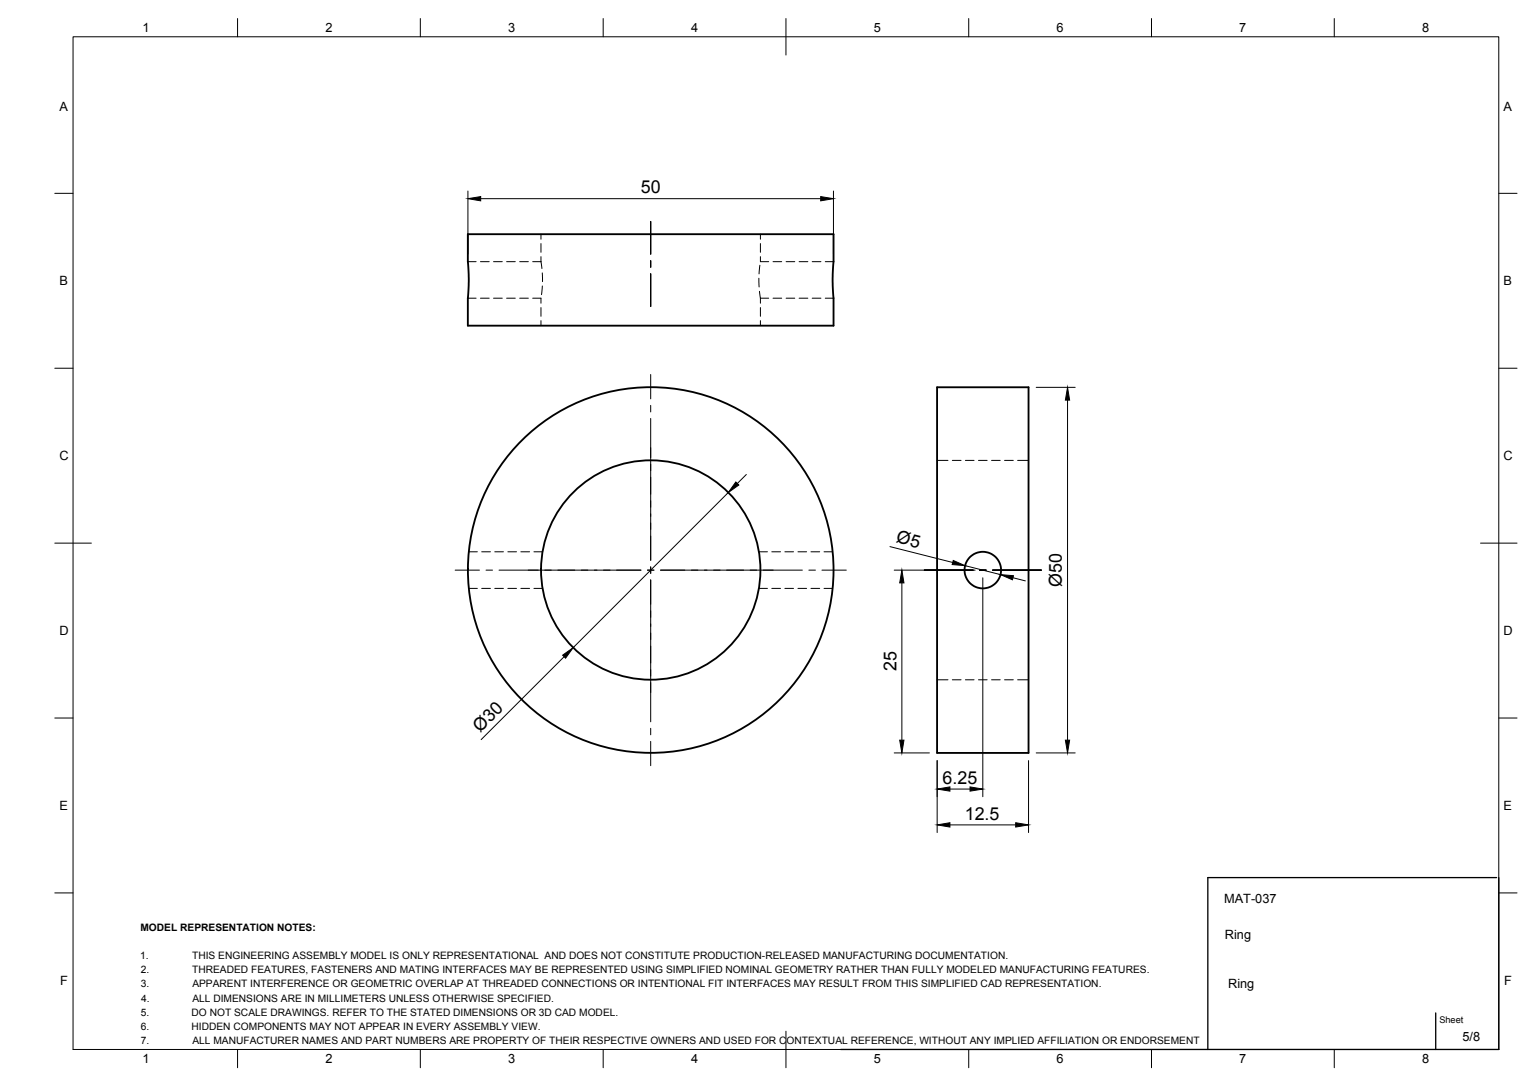
ISO-10303-21;
HEADER;
/* Generated by software containing ST-Developer
 * from STEP Tools, Inc. (www.steptools.com) 
 */

FILE_DESCRIPTION(
/* description */ ('STEP AP214'),
/* implementation_level */ '2;1');

FILE_NAME(
/* name */ 'ring.step',
/* time_stamp */ '2026-11-14T21:09:07-08:00',
/* author */ (''),
/* organization */ (''),
/* preprocessor_version */ 'ST-DEVELOPER v20.2',
/* originating_system */ 'Autodesk Translation Framework v15.17.0.0',
/* authorisation */ '');

FILE_SCHEMA (('AUTOMOTIVE_DESIGN { 1 0 10303 214 3 1 1 }'));
ENDSEC;

DATA;
#10=MECHANICAL_DESIGN_GEOMETRIC_PRESENTATION_REPRESENTATION('',(#81),#2059);
#67=SHAPE_REPRESENTATION_RELATIONSHIP('SRR','None',#2097,#74);
#74=ADVANCED_BREP_SHAPE_REPRESENTATION('',(#88),#2055);
#81=STYLED_ITEM('',(#2141),#88);
#88=MANIFOLD_SOLID_BREP('Body1',#978);
#112=PLANE('',#1135);
#113=PLANE('',#1136);
#139=FACE_BOUND('',#263,.T.);
#140=FACE_BOUND('',#264,.T.);
#141=FACE_BOUND('',#266,.T.);
#142=FACE_BOUND('',#267,.T.);
#143=FACE_BOUND('',#269,.T.);
#144=FACE_BOUND('',#271,.T.);
#149=B_SPLINE_CURVE_WITH_KNOTS('',3,(#1783,#1784,#1785,#1786,#1787,#1788,
#1789,#1790,#1791,#1792,#1793,#1794,#1795,#1796,#1797,#1798,#1799,#1800,
#1801,#1802,#1803,#1804,#1805,#1806,#1807,#1808,#1809,#1810,#1811,#1812,
#1813,#1814,#1815,#1816),.UNSPECIFIED.,.T.,.F.,(4,2,2,2,2,2,2,2,2,2,2,2,
2,2,2,2,4),(0.,0.0942394555075742,0.188478911015148,0.28271804575446,0.376957180493772,
0.471196315233084,0.565435449972396,0.65967490547997,0.753914360987544,
0.848153816495118,0.942393272002692,1.036632406742,1.13087154148132,1.22511067622063,
1.31934981095994,1.41358926646751,1.50782872197509),.UNSPECIFIED.);
#150=B_SPLINE_CURVE_WITH_KNOTS('',3,(#1820,#1821,#1822,#1823,#1824,#1825,
#1826,#1827,#1828,#1829,#1830,#1831,#1832,#1833,#1834,#1835,#1836,#1837),
 .UNSPECIFIED.,.F.,.F.,(4,2,2,2,2,2,2,2,4),(0.377444585314897,0.471804471485949,
0.566164357657001,0.660526764143398,0.754889170629794,0.849251577116191,
0.943613983602588,1.03797386977364,1.13233375594469),.UNSPECIFIED.);
#151=B_SPLINE_CURVE_WITH_KNOTS('',3,(#1838,#1839,#1840,#1841,#1842,#1843,
#1844,#1845,#1846,#1847,#1848,#1849,#1850,#1851,#1852,#1853,#1854,#1855,
#1856),.UNSPECIFIED.,.F.,.F.,(4,2,2,2,3,2,2,2,4),(-0.377444585314897,-0.283084699143845,
-0.188724812972793,-0.0943624064863967,0.,0.0943624064863968,0.188724812972794,
0.283084699143845,0.377444585314897),.UNSPECIFIED.);
#152=B_SPLINE_CURVE_WITH_KNOTS('',3,(#1860,#1861,#1862,#1863,#1864,#1865,
#1866,#1867,#1868,#1869,#1870,#1871,#1872,#1873,#1874,#1875,#1876,#1877),
 .UNSPECIFIED.,.F.,.F.,(4,2,2,2,2,2,2,2,4),(0.377444585314897,0.471804471485949,
0.566164357657001,0.660526764143397,0.754889170629794,0.849251577116191,
0.943613983602588,1.03797386977364,1.13233375594469),.UNSPECIFIED.);
#153=B_SPLINE_CURVE_WITH_KNOTS('',3,(#1880,#1881,#1882,#1883,#1884,#1885,
#1886,#1887,#1888,#1889,#1890,#1891,#1892,#1893,#1894,#1895,#1896,#1897,
#1898,#1899,#1900,#1901,#1902,#1903,#1904,#1905,#1906,#1907,#1908,#1909,
#1910,#1911,#1912,#1913),.UNSPECIFIED.,.T.,.F.,(4,2,2,2,2,2,2,2,2,2,2,2,
2,2,2,2,4),(-1.50782872197509,-1.41358926646751,-1.31934981095994,-1.22511067622063,
-1.13087154148132,-1.036632406742,-0.942393272002692,-0.848153816495118,
-0.753914360987544,-0.65967490547997,-0.565435449972396,-0.471196315233084,
-0.376957180493772,-0.28271804575446,-0.188478911015148,-0.0942394555075742,
0.),.UNSPECIFIED.);
#154=B_SPLINE_CURVE_WITH_KNOTS('',3,(#1914,#1915,#1916,#1917,#1918,#1919,
#1920,#1921,#1922,#1923,#1924,#1925,#1926,#1927,#1928,#1929,#1930,#1931,
#1932),.UNSPECIFIED.,.F.,.F.,(4,2,2,2,3,2,2,2,4),(1.13233375594469,1.22669364211574,
1.32105352828679,1.41541593477319,1.50977834125959,1.60414074774598,1.69850315423238,
1.79286304040343,1.88722292657449),.UNSPECIFIED.);
#190=FACE_OUTER_BOUND('',#260,.T.);
#191=FACE_OUTER_BOUND('',#261,.T.);
#192=FACE_OUTER_BOUND('',#262,.T.);
#193=FACE_OUTER_BOUND('',#265,.T.);
#194=FACE_OUTER_BOUND('',#268,.T.);
#195=FACE_OUTER_BOUND('',#270,.T.);
#260=EDGE_LOOP('',(#809,#810,#811,#812,#813));
#261=EDGE_LOOP('',(#814,#815,#816,#817,#818));
#262=EDGE_LOOP('',(#819,#820,#821,#822));
#263=EDGE_LOOP('',(#823,#824));
#264=EDGE_LOOP('',(#825,#826));
#265=EDGE_LOOP('',(#827,#828,#829,#830));
#266=EDGE_LOOP('',(#831));
#267=EDGE_LOOP('',(#832));
#268=EDGE_LOOP('',(#833));
#269=EDGE_LOOP('',(#834));
#270=EDGE_LOOP('',(#835));
#271=EDGE_LOOP('',(#836));
#331=LINE('',#1818,#396);
#332=LINE('',#1879,#397);
#333=LINE('',#1937,#398);
#334=LINE('',#1943,#399);
#396=VECTOR('',#1359,2.49999999999999);
#397=VECTOR('',#1362,2.49999999999999);
#398=VECTOR('',#1367,15.);
#399=VECTOR('',#1374,25.);
#446=CIRCLE('',#1130,15.);
#447=CIRCLE('',#1131,15.);
#448=CIRCLE('',#1133,25.);
#449=CIRCLE('',#1134,25.);
#510=VERTEX_POINT('',#1782);
#511=VERTEX_POINT('',#1817);
#512=VERTEX_POINT('',#1819);
#513=VERTEX_POINT('',#1858);
#514=VERTEX_POINT('',#1859);
#515=VERTEX_POINT('',#1878);
#516=VERTEX_POINT('',#1934);
#517=VERTEX_POINT('',#1936);
#518=VERTEX_POINT('',#1940);
#519=VERTEX_POINT('',#1942);
#615=EDGE_CURVE('',#510,#510,#149,.T.);
#616=EDGE_CURVE('',#510,#511,#331,.T.);
#617=EDGE_CURVE('',#511,#512,#150,.T.);
#618=EDGE_CURVE('',#512,#511,#151,.T.);
#619=EDGE_CURVE('',#513,#514,#152,.T.);
#620=EDGE_CURVE('',#514,#515,#332,.T.);
#621=EDGE_CURVE('',#515,#515,#153,.T.);
#622=EDGE_CURVE('',#514,#513,#154,.T.);
#623=EDGE_CURVE('',#516,#516,#446,.T.);
#624=EDGE_CURVE('',#516,#517,#333,.T.);
#625=EDGE_CURVE('',#517,#517,#447,.T.);
#626=EDGE_CURVE('',#518,#518,#448,.T.);
#627=EDGE_CURVE('',#518,#519,#334,.T.);
#628=EDGE_CURVE('',#519,#519,#449,.T.);
#809=ORIENTED_EDGE('',*,*,#615,.F.);
#810=ORIENTED_EDGE('',*,*,#616,.T.);
#811=ORIENTED_EDGE('',*,*,#617,.T.);
#812=ORIENTED_EDGE('',*,*,#618,.T.);
#813=ORIENTED_EDGE('',*,*,#616,.F.);
#814=ORIENTED_EDGE('',*,*,#619,.T.);
#815=ORIENTED_EDGE('',*,*,#620,.T.);
#816=ORIENTED_EDGE('',*,*,#621,.F.);
#817=ORIENTED_EDGE('',*,*,#620,.F.);
#818=ORIENTED_EDGE('',*,*,#622,.T.);
#819=ORIENTED_EDGE('',*,*,#623,.T.);
#820=ORIENTED_EDGE('',*,*,#624,.T.);
#821=ORIENTED_EDGE('',*,*,#625,.F.);
#822=ORIENTED_EDGE('',*,*,#624,.F.);
#823=ORIENTED_EDGE('',*,*,#619,.F.);
#824=ORIENTED_EDGE('',*,*,#622,.F.);
#825=ORIENTED_EDGE('',*,*,#618,.F.);
#826=ORIENTED_EDGE('',*,*,#617,.F.);
#827=ORIENTED_EDGE('',*,*,#626,.T.);
#828=ORIENTED_EDGE('',*,*,#627,.T.);
#829=ORIENTED_EDGE('',*,*,#628,.F.);
#830=ORIENTED_EDGE('',*,*,#627,.F.);
#831=ORIENTED_EDGE('',*,*,#615,.T.);
#832=ORIENTED_EDGE('',*,*,#621,.T.);
#833=ORIENTED_EDGE('',*,*,#628,.T.);
#834=ORIENTED_EDGE('',*,*,#623,.F.);
#835=ORIENTED_EDGE('',*,*,#626,.F.);
#836=ORIENTED_EDGE('',*,*,#625,.T.);
#910=CYLINDRICAL_SURFACE('',#1127,2.49999999999999);
#911=CYLINDRICAL_SURFACE('',#1128,2.49999999999999);
#912=CYLINDRICAL_SURFACE('',#1129,15.);
#913=CYLINDRICAL_SURFACE('',#1132,25.);
#953=ADVANCED_FACE('',(#190),#910,.F.);
#954=ADVANCED_FACE('',(#191),#911,.F.);
#955=ADVANCED_FACE('',(#192,#139,#140),#912,.F.);
#956=ADVANCED_FACE('',(#193,#141,#142),#913,.T.);
#957=ADVANCED_FACE('',(#194,#143),#112,.T.);
#958=ADVANCED_FACE('',(#195,#144),#113,.F.);
#978=CLOSED_SHELL('',(#953,#954,#955,#956,#957,#958));
#1126=AXIS2_PLACEMENT_3D('',#1780,#1355,#1356);
#1127=AXIS2_PLACEMENT_3D('',#1781,#1357,#1358);
#1128=AXIS2_PLACEMENT_3D('',#1857,#1360,#1361);
#1129=AXIS2_PLACEMENT_3D('',#1933,#1363,#1364);
#1130=AXIS2_PLACEMENT_3D('',#1935,#1365,#1366);
#1131=AXIS2_PLACEMENT_3D('',#1938,#1368,#1369);
#1132=AXIS2_PLACEMENT_3D('',#1939,#1370,#1371);
#1133=AXIS2_PLACEMENT_3D('',#1941,#1372,#1373);
#1134=AXIS2_PLACEMENT_3D('',#1944,#1375,#1376);
#1135=AXIS2_PLACEMENT_3D('',#1945,#1377,#1378);
#1136=AXIS2_PLACEMENT_3D('',#1946,#1379,#1380);
#1355=DIRECTION('axis',(0.,0.,1.));
#1356=DIRECTION('refdir',(1.,0.,0.));
#1357=DIRECTION('center_axis',(1.7347234759767E-18,1.,-1.38050658413677E-30));
#1358=DIRECTION('ref_axis',(-4.16000867987644E-29,1.38050658413677E-30,
1.));
#1359=DIRECTION('',(1.7347234759767E-18,1.,-1.38050658413677E-30));
#1360=DIRECTION('center_axis',(1.7347234759767E-18,1.,-1.38050658413677E-30));
#1361=DIRECTION('ref_axis',(-4.16000867987644E-29,1.38050658413677E-30,
1.));
#1362=DIRECTION('',(1.7347234759767E-18,1.,-1.38050658413677E-30));
#1363=DIRECTION('center_axis',(4.15754348954763E-29,4.93038065763134E-30,
-1.));
#1364=DIRECTION('ref_axis',(-1.,1.73472347598838E-18,-4.15754348954763E-29));
#1365=DIRECTION('center_axis',(-4.15754348954763E-29,-4.93038065763134E-30,
1.));
#1366=DIRECTION('ref_axis',(1.,-1.73472347598838E-18,4.15754348954763E-29));
#1367=DIRECTION('',(4.15754348954763E-29,4.93038065763134E-30,-1.));
#1368=DIRECTION('center_axis',(-4.15754348954763E-29,-4.93038065763134E-30,
1.));
#1369=DIRECTION('ref_axis',(1.,-1.73472347597692E-18,4.15754348954763E-29));
#1370=DIRECTION('center_axis',(4.15754348954763E-29,4.93038065763134E-30,
-1.));
#1371=DIRECTION('ref_axis',(-1.,1.73472347598312E-18,-4.15754348954763E-29));
#1372=DIRECTION('center_axis',(-4.15754348954763E-29,-4.93038065763134E-30,
1.));
#1373=DIRECTION('ref_axis',(1.,-1.73472347597692E-18,4.15754348954763E-29));
#1374=DIRECTION('',(-4.15754348954763E-29,-4.93038065763134E-30,1.));
#1375=DIRECTION('center_axis',(-4.15754348954763E-29,-4.93038065763134E-30,
1.));
#1376=DIRECTION('ref_axis',(1.,-1.73472347598312E-18,4.15754348954763E-29));
#1377=DIRECTION('center_axis',(4.1698694411917E-29,-4.93038065763134E-30,
1.));
#1378=DIRECTION('ref_axis',(1.,-1.73472347597692E-18,-4.1698694411917E-29));
#1379=DIRECTION('center_axis',(4.1698694411917E-29,-4.93038065763134E-30,
1.));
#1380=DIRECTION('ref_axis',(1.,-1.73472347597692E-18,-4.1698694411917E-29));
#1780=CARTESIAN_POINT('',(0.,0.,0.));
#1781=CARTESIAN_POINT('Origin',(-1.73472347597681E-15,-25.0000000000004,
6.24999999999996));
#1782=CARTESIAN_POINT('',(-1.42856179559609E-15,-25.0000000000024,3.74999999999996));
#1783=CARTESIAN_POINT('Ctrl Pts',(2.49999999999999,-24.8746859276679,6.24999999999996));
#1784=CARTESIAN_POINT('Ctrl Pts',(2.49999999999999,-24.8746859276679,5.93586848164138));
#1785=CARTESIAN_POINT('Ctrl Pts',(2.43717772293527,-24.8812496993573,5.6009428544044));
#1786=CARTESIAN_POINT('Ctrl Pts',(2.18197846805795,-24.9049270576873,4.98505712385862));
#1787=CARTESIAN_POINT('Ctrl Pts',(1.98961295362016,-24.9216954330504,4.7040790476874));
#1788=CARTESIAN_POINT('Ctrl Pts',(1.54592170742258,-24.9531478715761,4.26038780148982));
#1789=CARTESIAN_POINT('Ctrl Pts',(1.26494330018359,-24.9698795904327,4.06802169783962));
#1790=CARTESIAN_POINT('Ctrl Pts',(0.649056460774728,-24.9934730284172,3.81282200311052));
#1791=CARTESIAN_POINT('Ctrl Pts',(0.314130449131038,-25.0000000000024,3.74999999999997));
#1792=CARTESIAN_POINT('Ctrl Pts',(-0.314130449131041,-25.0000000000024,
3.74999999999997));
#1793=CARTESIAN_POINT('Ctrl Pts',(-0.649056460774731,-24.9934730284172,
3.81282200311052));
#1794=CARTESIAN_POINT('Ctrl Pts',(-1.26494330018359,-24.9698795904327,4.06802169783962));
#1795=CARTESIAN_POINT('Ctrl Pts',(-1.54592170742258,-24.9531478715761,4.26038780148982));
#1796=CARTESIAN_POINT('Ctrl Pts',(-1.98961295362016,-24.9216954330504,4.7040790476874));
#1797=CARTESIAN_POINT('Ctrl Pts',(-2.18197846805795,-24.9049270576873,4.98505712385862));
#1798=CARTESIAN_POINT('Ctrl Pts',(-2.43717772293527,-24.8812496993573,5.6009428544044));
#1799=CARTESIAN_POINT('Ctrl Pts',(-2.49999999999999,-24.8746859276679,5.93586848164138));
#1800=CARTESIAN_POINT('Ctrl Pts',(-2.49999999999999,-24.8746859276679,6.56413151835855));
#1801=CARTESIAN_POINT('Ctrl Pts',(-2.43717772293527,-24.8812496993573,6.89905714559553));
#1802=CARTESIAN_POINT('Ctrl Pts',(-2.18197846805795,-24.9049270576873,7.51494287614131));
#1803=CARTESIAN_POINT('Ctrl Pts',(-1.98961295362016,-24.9216954330504,7.79592095231253));
#1804=CARTESIAN_POINT('Ctrl Pts',(-1.54592170742258,-24.9531478715761,8.23961219851011));
#1805=CARTESIAN_POINT('Ctrl Pts',(-1.26494330018359,-24.9698795904327,8.43197830216031));
#1806=CARTESIAN_POINT('Ctrl Pts',(-0.649056460774732,-24.9934730284172,
8.68717799688941));
#1807=CARTESIAN_POINT('Ctrl Pts',(-0.314130449131042,-25.0000000000024,
8.74999999999996));
#1808=CARTESIAN_POINT('Ctrl Pts',(0.314130449131037,-25.0000000000024,8.74999999999996));
#1809=CARTESIAN_POINT('Ctrl Pts',(0.649056460774726,-24.9934730284172,8.68717799688941));
#1810=CARTESIAN_POINT('Ctrl Pts',(1.26494330018359,-24.9698795904327,8.43197830216031));
#1811=CARTESIAN_POINT('Ctrl Pts',(1.54592170742258,-24.9531478715761,8.23961219851011));
#1812=CARTESIAN_POINT('Ctrl Pts',(1.98961295362015,-24.9216954330504,7.79592095231254));
#1813=CARTESIAN_POINT('Ctrl Pts',(2.18197846805795,-24.9049270576873,7.51494287614131));
#1814=CARTESIAN_POINT('Ctrl Pts',(2.43717772293527,-24.8812496993573,6.89905714559553));
#1815=CARTESIAN_POINT('Ctrl Pts',(2.49999999999999,-24.8746859276679,6.56413151835855));
#1816=CARTESIAN_POINT('Ctrl Pts',(2.49999999999999,-24.8746859276679,6.24999999999996));
#1817=CARTESIAN_POINT('',(-2.15668646464658E-15,-15.0000000000024,3.74999999999997));
#1818=CARTESIAN_POINT('',(-2.04088517576354E-15,-25.0000000000004,3.74999999999997));
#1819=CARTESIAN_POINT('',(-1.73472347597681E-15,-14.9999999999981,8.74999999999997));
#1820=CARTESIAN_POINT('Ctrl Pts',(-2.22044604925031E-15,-15.0000000000024,
3.74999999999997));
#1821=CARTESIAN_POINT('Ctrl Pts',(-0.314532953903508,-15.0000000000024,
3.74999999999997));
#1822=CARTESIAN_POINT('Ctrl Pts',(-0.6496333501624,-14.989101375866,3.81297947750021));
#1823=CARTESIAN_POINT('Ctrl Pts',(-1.26541151060516,-14.9497129490456,4.0682974109409));
#1824=CARTESIAN_POINT('Ctrl Pts',(-1.54613758435442,-14.9217716767272,4.26060367842166));
#1825=CARTESIAN_POINT('Ctrl Pts',(-1.98940224121133,-14.8691658402789,4.70386833527857));
#1826=CARTESIAN_POINT('Ctrl Pts',(-2.18170386550859,-14.8410532029498,4.98459186762255));
#1827=CARTESIAN_POINT('Ctrl Pts',(-2.43701842756376,-14.8012713411841,5.60036129757765));
#1828=CARTESIAN_POINT('Ctrl Pts',(-2.49999999999999,-14.7901994577515,5.93545864504531));
#1829=CARTESIAN_POINT('Ctrl Pts',(-2.49999999999999,-14.7901994577515,6.56454135495462));
#1830=CARTESIAN_POINT('Ctrl Pts',(-2.43701842756376,-14.8012713411841,6.89963870242228));
#1831=CARTESIAN_POINT('Ctrl Pts',(-2.18170386550859,-14.8410532029498,7.51540813237737));
#1832=CARTESIAN_POINT('Ctrl Pts',(-1.98940224121133,-14.8691658402789,7.79613166472136));
#1833=CARTESIAN_POINT('Ctrl Pts',(-1.54613758435442,-14.9217716767272,8.23939632157827));
#1834=CARTESIAN_POINT('Ctrl Pts',(-1.26541151060516,-14.9497129490456,8.43170258905903));
#1835=CARTESIAN_POINT('Ctrl Pts',(-0.6496333501624,-14.989101375866,8.68702052249972));
#1836=CARTESIAN_POINT('Ctrl Pts',(-0.314532953903508,-15.0000000000024,
8.74999999999996));
#1837=CARTESIAN_POINT('Ctrl Pts',(-1.80411241501588E-15,-15.0000000000024,
8.74999999999996));
#1838=CARTESIAN_POINT('Ctrl Pts',(-1.80411241501588E-15,-15.0000000000024,
8.74999999999996));
#1839=CARTESIAN_POINT('Ctrl Pts',(0.314532953903504,-15.0000000000024,8.74999999999996));
#1840=CARTESIAN_POINT('Ctrl Pts',(0.649633350162397,-14.989101375866,8.68702052249972));
#1841=CARTESIAN_POINT('Ctrl Pts',(1.26541151060516,-14.9497129490456,8.43170258905903));
#1842=CARTESIAN_POINT('Ctrl Pts',(1.54613758435442,-14.9217716767272,8.23939632157827));
#1843=CARTESIAN_POINT('Ctrl Pts',(1.98940224121133,-14.8691658402789,7.79613166472136));
#1844=CARTESIAN_POINT('Ctrl Pts',(2.18170386550859,-14.8410532029498,7.51540813237737));
#1845=CARTESIAN_POINT('Ctrl Pts',(2.43701842756376,-14.8012713411841,6.89963870242228));
#1846=CARTESIAN_POINT('Ctrl Pts',(2.49999999999999,-14.7901994577515,6.56454135495462));
#1847=CARTESIAN_POINT('Ctrl Pts',(2.49999999999999,-14.7901994577515,6.24999999999996));
#1848=CARTESIAN_POINT('Ctrl Pts',(2.49999999999999,-14.7901994577515,5.93545864504531));
#1849=CARTESIAN_POINT('Ctrl Pts',(2.43701842756376,-14.8012713411841,5.60036129757765));
#1850=CARTESIAN_POINT('Ctrl Pts',(2.18170386550859,-14.8410532029498,4.98459186762255));
#1851=CARTESIAN_POINT('Ctrl Pts',(1.98940224121133,-14.8691658402789,4.70386833527857));
#1852=CARTESIAN_POINT('Ctrl Pts',(1.54613758435442,-14.9217716767272,4.26060367842166));
#1853=CARTESIAN_POINT('Ctrl Pts',(1.26541151060516,-14.9497129490456,4.0682974109409));
#1854=CARTESIAN_POINT('Ctrl Pts',(0.649633350162397,-14.989101375866,3.81297947750021));
#1855=CARTESIAN_POINT('Ctrl Pts',(0.314532953903504,-15.0000000000024,3.74999999999997));
#1856=CARTESIAN_POINT('Ctrl Pts',(-2.28983498828939E-15,-15.0000000000024,
3.74999999999997));
#1857=CARTESIAN_POINT('Origin',(-1.73472347597681E-15,-25.0000000000004,
6.24999999999996));
#1858=CARTESIAN_POINT('',(-1.73472347597681E-15,15.0000000000001,8.74999999999997));
#1859=CARTESIAN_POINT('',(-1.67963750875296E-15,14.9999999999975,3.74999999999997));
#1860=CARTESIAN_POINT('Ctrl Pts',(-2.22044604925031E-15,14.9999999999975,
8.74999999999996));
#1861=CARTESIAN_POINT('Ctrl Pts',(-0.314532953903508,14.9999999999975,8.74999999999996));
#1862=CARTESIAN_POINT('Ctrl Pts',(-0.6496333501624,14.9891013758612,8.68702052249972));
#1863=CARTESIAN_POINT('Ctrl Pts',(-1.26541151060517,14.9497129490408,8.43170258905903));
#1864=CARTESIAN_POINT('Ctrl Pts',(-1.54613758435443,14.9217716767223,8.23939632157827));
#1865=CARTESIAN_POINT('Ctrl Pts',(-1.98940224121133,14.869165840274,7.79613166472136));
#1866=CARTESIAN_POINT('Ctrl Pts',(-2.18170386550859,14.841053202945,7.51540813237737));
#1867=CARTESIAN_POINT('Ctrl Pts',(-2.43701842756376,14.8012713411792,6.89963870242228));
#1868=CARTESIAN_POINT('Ctrl Pts',(-2.49999999999999,14.7901994577466,6.56454135495462));
#1869=CARTESIAN_POINT('Ctrl Pts',(-2.49999999999999,14.7901994577466,5.93545864504531));
#1870=CARTESIAN_POINT('Ctrl Pts',(-2.43701842756376,14.8012713411792,5.60036129757765));
#1871=CARTESIAN_POINT('Ctrl Pts',(-2.18170386550859,14.841053202945,4.98459186762255));
#1872=CARTESIAN_POINT('Ctrl Pts',(-1.98940224121133,14.869165840274,4.70386833527857));
#1873=CARTESIAN_POINT('Ctrl Pts',(-1.54613758435442,14.9217716767223,4.26060367842166));
#1874=CARTESIAN_POINT('Ctrl Pts',(-1.26541151060516,14.9497129490408,4.0682974109409));
#1875=CARTESIAN_POINT('Ctrl Pts',(-0.649633350162399,14.9891013758612,3.81297947750021));
#1876=CARTESIAN_POINT('Ctrl Pts',(-0.314532953903507,14.9999999999975,3.74999999999997));
#1877=CARTESIAN_POINT('Ctrl Pts',(-1.2490009027033E-15,14.9999999999975,
3.74999999999997));
#1878=CARTESIAN_POINT('',(-1.34182558298458E-15,24.9999999999976,3.74999999999996));
#1879=CARTESIAN_POINT('',(-2.04088517576354E-15,-25.0000000000004,3.74999999999997));
#1880=CARTESIAN_POINT('Ctrl Pts',(2.49999999999999,24.874685927663,6.24999999999996));
#1881=CARTESIAN_POINT('Ctrl Pts',(2.49999999999999,24.874685927663,6.56413151835855));
#1882=CARTESIAN_POINT('Ctrl Pts',(2.43717772293527,24.8812496993524,6.89905714559553));
#1883=CARTESIAN_POINT('Ctrl Pts',(2.18197846805795,24.9049270576824,7.51494287614131));
#1884=CARTESIAN_POINT('Ctrl Pts',(1.98961295362016,24.9216954330456,7.79592095231253));
#1885=CARTESIAN_POINT('Ctrl Pts',(1.54592170742258,24.9531478715712,8.23961219851011));
#1886=CARTESIAN_POINT('Ctrl Pts',(1.26494330018359,24.9698795904278,8.43197830216031));
#1887=CARTESIAN_POINT('Ctrl Pts',(0.649056460774728,24.9934730284123,8.68717799688941));
#1888=CARTESIAN_POINT('Ctrl Pts',(0.314130449131038,24.9999999999975,8.74999999999996));
#1889=CARTESIAN_POINT('Ctrl Pts',(-0.314130449131041,24.9999999999975,8.74999999999996));
#1890=CARTESIAN_POINT('Ctrl Pts',(-0.649056460774732,24.9934730284123,8.68717799688941));
#1891=CARTESIAN_POINT('Ctrl Pts',(-1.26494330018359,24.9698795904278,8.43197830216031));
#1892=CARTESIAN_POINT('Ctrl Pts',(-1.54592170742258,24.9531478715712,8.23961219851011));
#1893=CARTESIAN_POINT('Ctrl Pts',(-1.98961295362016,24.9216954330456,7.79592095231253));
#1894=CARTESIAN_POINT('Ctrl Pts',(-2.18197846805795,24.9049270576824,7.51494287614131));
#1895=CARTESIAN_POINT('Ctrl Pts',(-2.43717772293527,24.8812496993524,6.89905714559553));
#1896=CARTESIAN_POINT('Ctrl Pts',(-2.49999999999999,24.874685927663,6.56413151835855));
#1897=CARTESIAN_POINT('Ctrl Pts',(-2.49999999999999,24.874685927663,5.93586848164138));
#1898=CARTESIAN_POINT('Ctrl Pts',(-2.43717772293527,24.8812496993524,5.6009428544044));
#1899=CARTESIAN_POINT('Ctrl Pts',(-2.18197846805795,24.9049270576824,4.98505712385862));
#1900=CARTESIAN_POINT('Ctrl Pts',(-1.98961295362016,24.9216954330456,4.7040790476874));
#1901=CARTESIAN_POINT('Ctrl Pts',(-1.54592170742258,24.9531478715712,4.26038780148982));
#1902=CARTESIAN_POINT('Ctrl Pts',(-1.26494330018359,24.9698795904278,4.06802169783962));
#1903=CARTESIAN_POINT('Ctrl Pts',(-0.649056460774731,24.9934730284123,3.81282200311052));
#1904=CARTESIAN_POINT('Ctrl Pts',(-0.314130449131041,24.9999999999975,3.74999999999997));
#1905=CARTESIAN_POINT('Ctrl Pts',(0.314130449131038,24.9999999999975,3.74999999999997));
#1906=CARTESIAN_POINT('Ctrl Pts',(0.649056460774727,24.9934730284123,3.81282200311052));
#1907=CARTESIAN_POINT('Ctrl Pts',(1.26494330018359,24.9698795904278,4.06802169783962));
#1908=CARTESIAN_POINT('Ctrl Pts',(1.54592170742258,24.9531478715712,4.26038780148982));
#1909=CARTESIAN_POINT('Ctrl Pts',(1.98961295362016,24.9216954330456,4.7040790476874));
#1910=CARTESIAN_POINT('Ctrl Pts',(2.18197846805795,24.9049270576824,4.98505712385862));
#1911=CARTESIAN_POINT('Ctrl Pts',(2.43717772293527,24.8812496993524,5.6009428544044));
#1912=CARTESIAN_POINT('Ctrl Pts',(2.49999999999999,24.874685927663,5.93586848164138));
#1913=CARTESIAN_POINT('Ctrl Pts',(2.49999999999999,24.874685927663,6.24999999999996));
#1914=CARTESIAN_POINT('Ctrl Pts',(-1.31838984174237E-15,14.9999999999975,
3.74999999999997));
#1915=CARTESIAN_POINT('Ctrl Pts',(0.314532953903505,14.9999999999975,3.74999999999997));
#1916=CARTESIAN_POINT('Ctrl Pts',(0.649633350162396,14.9891013758612,3.81297947750021));
#1917=CARTESIAN_POINT('Ctrl Pts',(1.26541151060516,14.9497129490408,4.0682974109409));
#1918=CARTESIAN_POINT('Ctrl Pts',(1.54613758435442,14.9217716767223,4.26060367842166));
#1919=CARTESIAN_POINT('Ctrl Pts',(1.98940224121133,14.869165840274,4.70386833527857));
#1920=CARTESIAN_POINT('Ctrl Pts',(2.18170386550859,14.841053202945,4.98459186762255));
#1921=CARTESIAN_POINT('Ctrl Pts',(2.43701842756376,14.8012713411792,5.60036129757765));
#1922=CARTESIAN_POINT('Ctrl Pts',(2.49999999999999,14.7901994577466,5.93545864504531));
#1923=CARTESIAN_POINT('Ctrl Pts',(2.49999999999999,14.7901994577466,6.24999999999996));
#1924=CARTESIAN_POINT('Ctrl Pts',(2.49999999999999,14.7901994577466,6.56454135495462));
#1925=CARTESIAN_POINT('Ctrl Pts',(2.43701842756376,14.8012713411792,6.89963870242228));
#1926=CARTESIAN_POINT('Ctrl Pts',(2.18170386550859,14.841053202945,7.51540813237737));
#1927=CARTESIAN_POINT('Ctrl Pts',(1.98940224121133,14.869165840274,7.79613166472136));
#1928=CARTESIAN_POINT('Ctrl Pts',(1.54613758435442,14.9217716767223,8.23939632157827));
#1929=CARTESIAN_POINT('Ctrl Pts',(1.26541151060516,14.9497129490408,8.43170258905903));
#1930=CARTESIAN_POINT('Ctrl Pts',(0.649633350162395,14.9891013758612,8.68702052249972));
#1931=CARTESIAN_POINT('Ctrl Pts',(0.314532953903504,14.9999999999975,8.74999999999996));
#1932=CARTESIAN_POINT('Ctrl Pts',(-2.22044604925031E-15,14.9999999999975,
8.74999999999996));
#1933=CARTESIAN_POINT('Origin',(-1.73472347597681E-15,-2.44249065417534E-12,
12.5));
#1934=CARTESIAN_POINT('',(15.,-2.44435364522621E-12,12.5));
#1935=CARTESIAN_POINT('Origin',(-1.73472347597681E-15,-2.44249065417534E-12,
12.5));
#1936=CARTESIAN_POINT('',(15.,-2.44435364522621E-12,0.));
#1937=CARTESIAN_POINT('',(15.,-2.44435364522621E-12,12.5));
#1938=CARTESIAN_POINT('Origin',(0.,0.,0.));
#1939=CARTESIAN_POINT('Origin',(-1.73472347597681E-15,-2.44249065417534E-12,
12.5));
#1940=CARTESIAN_POINT('',(25.,-2.44559563926011E-12,2.22044604925031E-15));
#1941=CARTESIAN_POINT('Origin',(0.,0.,0.));
#1942=CARTESIAN_POINT('',(25.,-2.44559563926011E-12,12.5));
#1943=CARTESIAN_POINT('',(25.,-2.44559563926011E-12,12.5));
#1944=CARTESIAN_POINT('Origin',(-1.73472347597681E-15,-2.44249065417534E-12,
12.5));
#1945=CARTESIAN_POINT('Origin',(-1.73472347597681E-15,-2.44249065417534E-12,
12.5));
#1946=CARTESIAN_POINT('Origin',(0.,0.,0.));
#2046=UNCERTAINTY_MEASURE_WITH_UNIT(LENGTH_MEASURE(0.01),#2060,
'DISTANCE_ACCURACY_VALUE',
'Maximum model space distance between geometric entities at asserted c
onnectivities');
#2050=UNCERTAINTY_MEASURE_WITH_UNIT(LENGTH_MEASURE(0.01),#2060,
'DISTANCE_ACCURACY_VALUE',
'Maximum model space distance between geometric entities at asserted c
onnectivities');
#2055=(
GEOMETRIC_REPRESENTATION_CONTEXT(3)
GLOBAL_UNCERTAINTY_ASSIGNED_CONTEXT((#2046))
GLOBAL_UNIT_ASSIGNED_CONTEXT((#2060,#2062,#2063))
REPRESENTATION_CONTEXT('','3D')
);
#2059=(
GEOMETRIC_REPRESENTATION_CONTEXT(3)
GLOBAL_UNCERTAINTY_ASSIGNED_CONTEXT((#2050))
GLOBAL_UNIT_ASSIGNED_CONTEXT((#2060,#2062,#2063))
REPRESENTATION_CONTEXT('','3D')
);
#2060=(
LENGTH_UNIT()
NAMED_UNIT(*)
SI_UNIT(.MILLI.,.METRE.)
);
#2062=(
NAMED_UNIT(*)
PLANE_ANGLE_UNIT()
SI_UNIT($,.RADIAN.)
);
#2063=(
NAMED_UNIT(*)
SI_UNIT($,.STERADIAN.)
SOLID_ANGLE_UNIT()
);
#2068=SHAPE_DEFINITION_REPRESENTATION(#2076,#2097);
#2076=PRODUCT_DEFINITION_SHAPE('',$,#2106);
#2097=SHAPE_REPRESENTATION('',(#1126),#2055);
#2101=PRODUCT_DEFINITION_CONTEXT('part definition',#2127,'design');
#2106=PRODUCT_DEFINITION('Ring','ring',#2114,#2101);
#2114=PRODUCT_DEFINITION_FORMATION('',$,#2133);
#2127=APPLICATION_CONTEXT(
'Core Data for Automotive Mechanical Design Process');
#2128=PRODUCT_CONTEXT('part definition',#2127,'mechanical');
#2133=PRODUCT('Ring','ring',$,(#2128));
#2141=PRESENTATION_STYLE_ASSIGNMENT((#2147));
#2147=SURFACE_STYLE_USAGE(.BOTH.,#2153);
#2153=SURFACE_SIDE_STYLE('',(#2159));
#2159=SURFACE_STYLE_FILL_AREA(#2165);
#2165=FILL_AREA_STYLE('Opaque(97,158,199)',(#2171));
#2171=FILL_AREA_STYLE_COLOUR('Opaque(97,158,199)',#2177);
#2177=COLOUR_RGB('Opaque(97,158,199)',0.380392156862745,0.619607843137255,
0.780392156862745);
ENDSEC;
END-ISO-10303-21;
